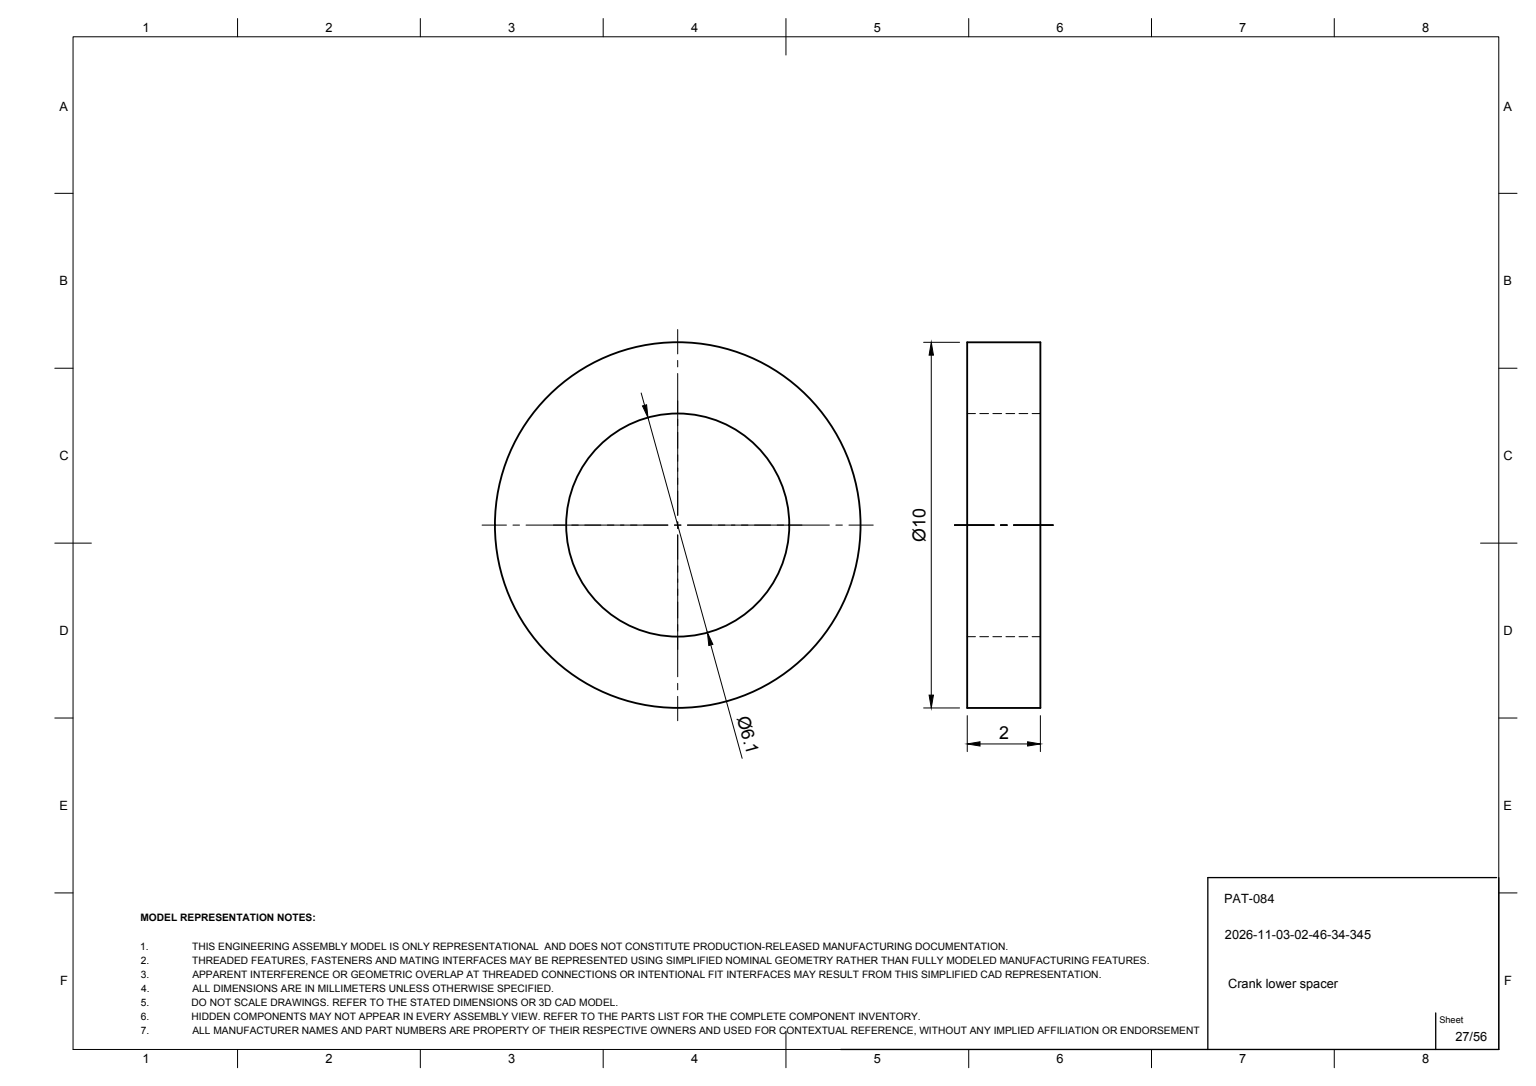
ISO-10303-21;
HEADER;
/* Generated by software containing ST-Developer
 * from STEP Tools, Inc. (www.steptools.com) 
 */

FILE_DESCRIPTION(
/* description */ ('Quick-return (Whitworth) mechanism'),
/* implementation_level */ '2;1');

FILE_NAME(
/* name */ 'Crank lower spacer.step',
/* time_stamp */ '2026-10-28T03:25:57-07:00',
/* author */ (''),
/* organization */ (''),
/* preprocessor_version */ 'ST-DEVELOPER v20.2',
/* originating_system */ 'Autodesk Translation Framework v15.17.0.0',
/* authorisation */ '');

FILE_SCHEMA (('AUTOMOTIVE_DESIGN { 1 0 10303 214 3 1 1 }'));
ENDSEC;

DATA;
#10=MECHANICAL_DESIGN_GEOMETRIC_PRESENTATION_REPRESENTATION('',(#516),#14878);
#420=SHAPE_REPRESENTATION_RELATIONSHIP('SRR','None',#15090,#464);
#464=ADVANCED_BREP_SHAPE_REPRESENTATION('',(#568),#14847);
#516=STYLED_ITEM('',(#15420),#568);
#568=MANIFOLD_SOLID_BREP('Body1',#7870);
#718=FACE_BOUND('',#1885,.T.);
#719=FACE_BOUND('',#1887,.T.);
#895=PLANE('',#8934);
#896=PLANE('',#8935);
#1289=FACE_OUTER_BOUND('',#1882,.T.);
#1290=FACE_OUTER_BOUND('',#1883,.T.);
#1291=FACE_OUTER_BOUND('',#1884,.T.);
#1292=FACE_OUTER_BOUND('',#1886,.T.);
#1882=EDGE_LOOP('',(#6282,#6283,#6284,#6285));
#1883=EDGE_LOOP('',(#6286,#6287,#6288,#6289));
#1884=EDGE_LOOP('',(#6290));
#1885=EDGE_LOOP('',(#6291));
#1886=EDGE_LOOP('',(#6292));
#1887=EDGE_LOOP('',(#6293));
#2375=LINE('',#13616,#2898);
#2376=LINE('',#13622,#2899);
#2898=VECTOR('',#10694,0.305);
#2899=VECTOR('',#10701,0.5);
#3490=CIRCLE('',#8929,0.305);
#3491=CIRCLE('',#8930,0.305);
#3492=CIRCLE('',#8932,0.5);
#3493=CIRCLE('',#8933,0.5);
#3982=VERTEX_POINT('',#13613);
#3983=VERTEX_POINT('',#13615);
#3984=VERTEX_POINT('',#13619);
#3985=VERTEX_POINT('',#13621);
#4798=EDGE_CURVE('',#3982,#3982,#3490,.T.);
#4799=EDGE_CURVE('',#3982,#3983,#2375,.T.);
#4800=EDGE_CURVE('',#3983,#3983,#3491,.T.);
#4801=EDGE_CURVE('',#3984,#3984,#3492,.T.);
#4802=EDGE_CURVE('',#3984,#3985,#2376,.T.);
#4803=EDGE_CURVE('',#3985,#3985,#3493,.T.);
#6282=ORIENTED_EDGE('',*,*,#4798,.F.);
#6283=ORIENTED_EDGE('',*,*,#4799,.T.);
#6284=ORIENTED_EDGE('',*,*,#4800,.T.);
#6285=ORIENTED_EDGE('',*,*,#4799,.F.);
#6286=ORIENTED_EDGE('',*,*,#4801,.F.);
#6287=ORIENTED_EDGE('',*,*,#4802,.T.);
#6288=ORIENTED_EDGE('',*,*,#4803,.T.);
#6289=ORIENTED_EDGE('',*,*,#4802,.F.);
#6290=ORIENTED_EDGE('',*,*,#4801,.T.);
#6291=ORIENTED_EDGE('',*,*,#4798,.T.);
#6292=ORIENTED_EDGE('',*,*,#4803,.F.);
#6293=ORIENTED_EDGE('',*,*,#4800,.F.);
#7317=CYLINDRICAL_SURFACE('',#8928,0.305);
#7318=CYLINDRICAL_SURFACE('',#8931,0.5);
#7620=ADVANCED_FACE('',(#1289),#7317,.F.);
#7621=ADVANCED_FACE('',(#1290),#7318,.T.);
#7622=ADVANCED_FACE('',(#1291,#718),#895,.T.);
#7623=ADVANCED_FACE('',(#1292,#719),#896,.F.);
#7870=CLOSED_SHELL('',(#7620,#7621,#7622,#7623));
#8927=AXIS2_PLACEMENT_3D('',#13611,#10688,#10689);
#8928=AXIS2_PLACEMENT_3D('',#13612,#10690,#10691);
#8929=AXIS2_PLACEMENT_3D('',#13614,#10692,#10693);
#8930=AXIS2_PLACEMENT_3D('',#13617,#10695,#10696);
#8931=AXIS2_PLACEMENT_3D('',#13618,#10697,#10698);
#8932=AXIS2_PLACEMENT_3D('',#13620,#10699,#10700);
#8933=AXIS2_PLACEMENT_3D('',#13623,#10702,#10703);
#8934=AXIS2_PLACEMENT_3D('',#13624,#10704,#10705);
#8935=AXIS2_PLACEMENT_3D('',#13625,#10706,#10707);
#10688=DIRECTION('axis',(0.,0.,1.));
#10689=DIRECTION('refdir',(1.,0.,0.));
#10690=DIRECTION('center_axis',(0.,0.,1.));
#10691=DIRECTION('ref_axis',(1.,0.,0.));
#10692=DIRECTION('center_axis',(0.,0.,-1.));
#10693=DIRECTION('ref_axis',(1.,0.,0.));
#10694=DIRECTION('',(0.,0.,-1.));
#10695=DIRECTION('center_axis',(0.,0.,-1.));
#10696=DIRECTION('ref_axis',(1.,0.,0.));
#10697=DIRECTION('center_axis',(0.,0.,1.));
#10698=DIRECTION('ref_axis',(1.,0.,0.));
#10699=DIRECTION('center_axis',(0.,0.,1.));
#10700=DIRECTION('ref_axis',(1.,0.,0.));
#10701=DIRECTION('',(0.,0.,-1.));
#10702=DIRECTION('center_axis',(0.,0.,1.));
#10703=DIRECTION('ref_axis',(1.,0.,0.));
#10704=DIRECTION('center_axis',(0.,0.,1.));
#10705=DIRECTION('ref_axis',(1.,0.,0.));
#10706=DIRECTION('center_axis',(0.,0.,1.));
#10707=DIRECTION('ref_axis',(1.,0.,0.));
#13611=CARTESIAN_POINT('',(0.,0.,0.));
#13612=CARTESIAN_POINT('Origin',(0.,9.,6.));
#13613=CARTESIAN_POINT('',(-0.305,9.,6.2));
#13614=CARTESIAN_POINT('Origin',(0.,9.,6.2));
#13615=CARTESIAN_POINT('',(-0.305,9.,6.));
#13616=CARTESIAN_POINT('',(-0.305,9.,6.));
#13617=CARTESIAN_POINT('Origin',(0.,9.,6.));
#13618=CARTESIAN_POINT('Origin',(0.,9.,6.));
#13619=CARTESIAN_POINT('',(-0.5,9.,6.2));
#13620=CARTESIAN_POINT('Origin',(0.,9.,6.2));
#13621=CARTESIAN_POINT('',(-0.5,9.,6.));
#13622=CARTESIAN_POINT('',(-0.5,9.,6.));
#13623=CARTESIAN_POINT('Origin',(0.,9.,6.));
#13624=CARTESIAN_POINT('Origin',(0.,9.,6.2));
#13625=CARTESIAN_POINT('Origin',(0.,9.,6.));
#14793=UNCERTAINTY_MEASURE_WITH_UNIT(LENGTH_MEASURE(0.001),#14879,
'DISTANCE_ACCURACY_VALUE',
'Maximum model space distance between geometric entities at asserted c
onnectivities');
#14824=UNCERTAINTY_MEASURE_WITH_UNIT(LENGTH_MEASURE(0.001),#14879,
'DISTANCE_ACCURACY_VALUE',
'Maximum model space distance between geometric entities at asserted c
onnectivities');
#14847=(
GEOMETRIC_REPRESENTATION_CONTEXT(3)
GLOBAL_UNCERTAINTY_ASSIGNED_CONTEXT((#14793))
GLOBAL_UNIT_ASSIGNED_CONTEXT((#14879,#14881,#14882))
REPRESENTATION_CONTEXT('','3D')
);
#14878=(
GEOMETRIC_REPRESENTATION_CONTEXT(3)
GLOBAL_UNCERTAINTY_ASSIGNED_CONTEXT((#14824))
GLOBAL_UNIT_ASSIGNED_CONTEXT((#14879,#14881,#14882))
REPRESENTATION_CONTEXT('','3D')
);
#14879=(
LENGTH_UNIT()
NAMED_UNIT(*)
SI_UNIT(.CENTI.,.METRE.)
);
#14881=(
NAMED_UNIT(*)
PLANE_ANGLE_UNIT()
SI_UNIT($,.RADIAN.)
);
#14882=(
NAMED_UNIT(*)
SI_UNIT($,.STERADIAN.)
SOLID_ANGLE_UNIT()
);
#14905=SHAPE_DEFINITION_REPRESENTATION(#14963,#15090);
#14963=PRODUCT_DEFINITION_SHAPE('',$,#15144);
#15090=SHAPE_REPRESENTATION('',(#8927),#14847);
#15121=PRODUCT_DEFINITION_CONTEXT('part definition',#15282,'design');
#15144=PRODUCT_DEFINITION('Crank lower spacer','Crank lower spacer',#15197,
#15121);
#15197=PRODUCT_DEFINITION_FORMATION('',$,#15306);
#15282=APPLICATION_CONTEXT(
'Core Data for Automotive Mechanical Design Process');
#15283=PRODUCT_CONTEXT('part definition',#15282,'mechanical');
#15306=PRODUCT('Crank lower spacer','Crank lower spacer',
'Crank lower spacer',(#15283));
#15414=COLOUR_RGB('Off White',0.89,0.88,0.83);
#15415=FILL_AREA_STYLE_COLOUR('',#15414);
#15416=FILL_AREA_STYLE('',(#15415));
#15417=SURFACE_STYLE_FILL_AREA(#15416);
#15418=SURFACE_SIDE_STYLE('',(#15417));
#15419=SURFACE_STYLE_USAGE(.BOTH.,#15418);
#15420=PRESENTATION_STYLE_ASSIGNMENT((#15419));
ENDSEC;
END-ISO-10303-21;
